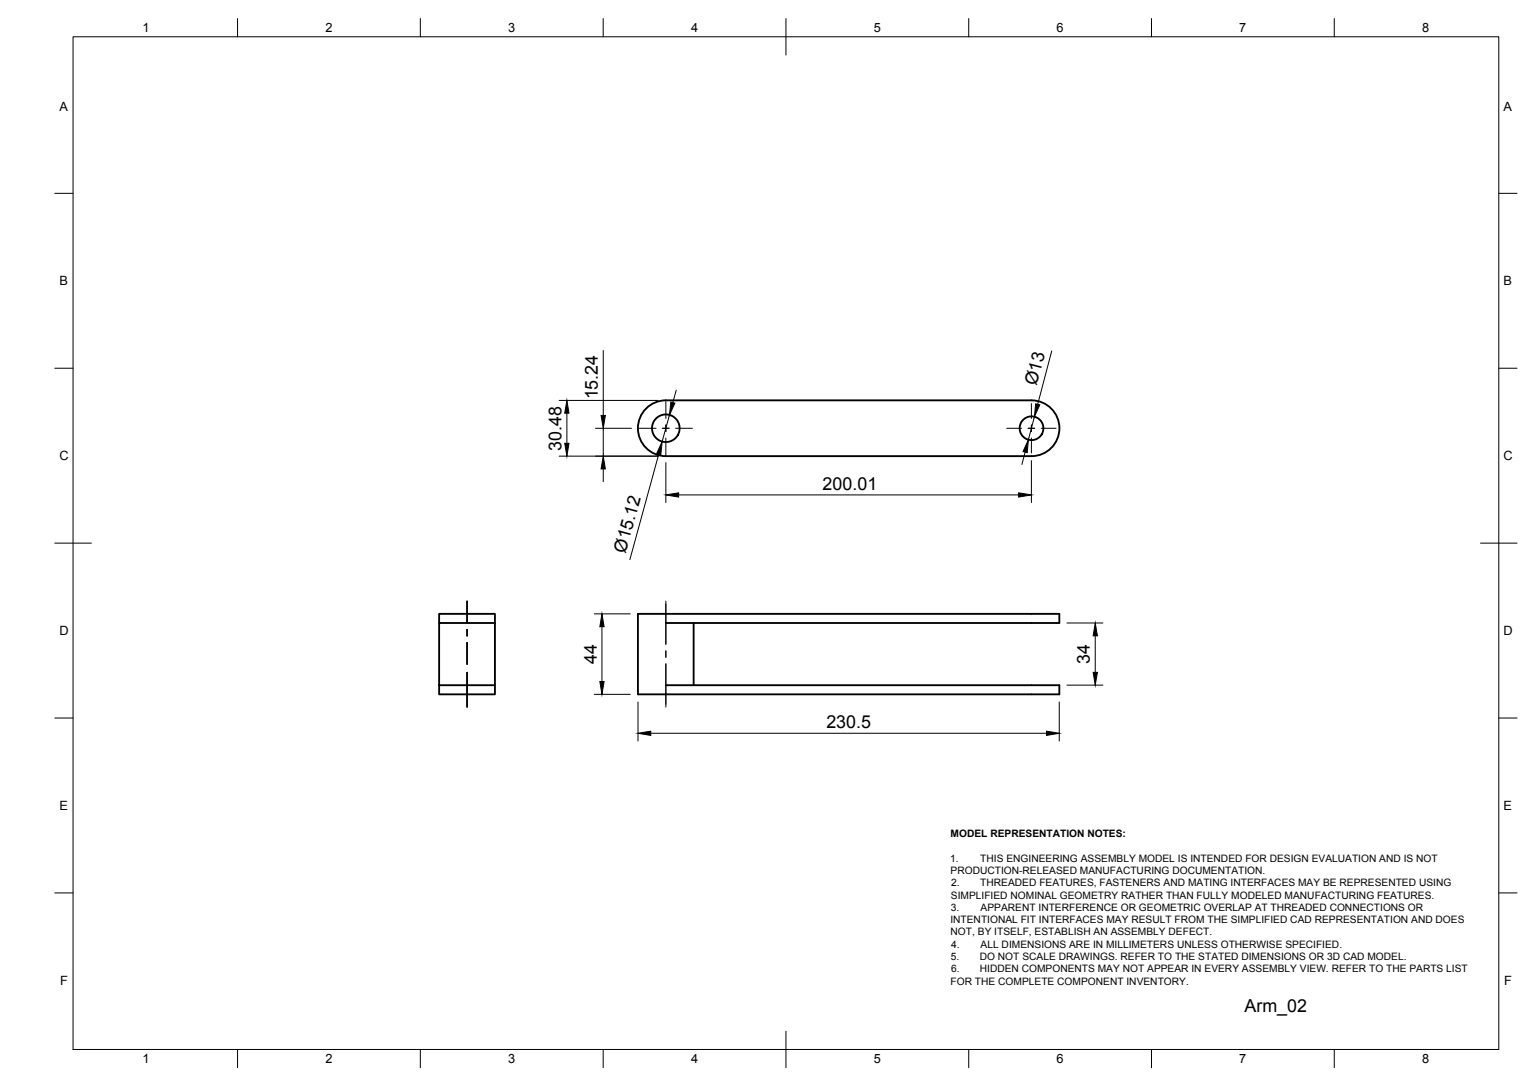
ISO-10303-21;
HEADER;
/* Generated by software containing ST-Developer
 * from STEP Tools, Inc. (www.steptools.com) 
 */

FILE_DESCRIPTION(
/* description */ (''),
/* implementation_level */ '2;1');

FILE_NAME(
/* name */ 'Arm_02.step',
/* time_stamp */ '2026-10-06T13:41:14-07:00',
/* author */ (''),
/* organization */ (''),
/* preprocessor_version */ 'ST-DEVELOPER v20.2',
/* originating_system */ 'Autodesk Translation Framework v15.15.0.0',
/* authorisation */ '');

FILE_SCHEMA (('AUTOMOTIVE_DESIGN { 1 0 10303 214 3 1 1 }'));
ENDSEC;

DATA;
#10=MECHANICAL_DESIGN_GEOMETRIC_PRESENTATION_REPRESENTATION('',(#1968),#279266);
#1950=SHAPE_REPRESENTATION_RELATIONSHIP('SRR','None',#279309,#1959);
#1959=ADVANCED_BREP_SHAPE_REPRESENTATION('',(#1977),#279265);
#1968=STYLED_ITEM('',(#279355),#1977);
#1977=MANIFOLD_SOLID_BREP('Body1',#14946);
#2018=FACE_BOUND('',#3081,.T.);
#2019=FACE_BOUND('',#3083,.T.);
#2020=FACE_BOUND('',#3084,.T.);
#2021=FACE_BOUND('',#3092,.T.);
#2022=FACE_BOUND('',#3094,.T.);
#2023=FACE_BOUND('',#3095,.T.);
#2102=PLANE('',#15640);
#2103=PLANE('',#15644);
#2104=PLANE('',#15645);
#2105=PLANE('',#15647);
#2106=PLANE('',#15655);
#2107=PLANE('',#15659);
#2108=PLANE('',#15663);
#2109=PLANE('',#15664);
#2566=FACE_OUTER_BOUND('',#3076,.T.);
#2567=FACE_OUTER_BOUND('',#3077,.T.);
#2568=FACE_OUTER_BOUND('',#3078,.T.);
#2569=FACE_OUTER_BOUND('',#3079,.T.);
#2570=FACE_OUTER_BOUND('',#3080,.T.);
#2571=FACE_OUTER_BOUND('',#3082,.T.);
#2572=FACE_OUTER_BOUND('',#3085,.T.);
#2573=FACE_OUTER_BOUND('',#3086,.T.);
#2574=FACE_OUTER_BOUND('',#3087,.T.);
#2575=FACE_OUTER_BOUND('',#3088,.T.);
#2576=FACE_OUTER_BOUND('',#3089,.T.);
#2577=FACE_OUTER_BOUND('',#3090,.T.);
#2578=FACE_OUTER_BOUND('',#3091,.T.);
#2579=FACE_OUTER_BOUND('',#3093,.T.);
#3076=EDGE_LOOP('',(#14026,#14027,#14028,#14029));
#3077=EDGE_LOOP('',(#14030,#14031,#14032,#14033));
#3078=EDGE_LOOP('',(#14034,#14035,#14036,#14037));
#3079=EDGE_LOOP('',(#14038,#14039,#14040,#14041));
#3080=EDGE_LOOP('',(#14042,#14043,#14044,#14045));
#3081=EDGE_LOOP('',(#14046));
#3082=EDGE_LOOP('',(#14047,#14048,#14049,#14050));
#3083=EDGE_LOOP('',(#14051));
#3084=EDGE_LOOP('',(#14052));
#3085=EDGE_LOOP('',(#14053,#14054,#14055,#14056));
#3086=EDGE_LOOP('',(#14057,#14058,#14059,#14060));
#3087=EDGE_LOOP('',(#14061,#14062,#14063,#14064));
#3088=EDGE_LOOP('',(#14065,#14066,#14067,#14068));
#3089=EDGE_LOOP('',(#14069,#14070,#14071,#14072));
#3090=EDGE_LOOP('',(#14073,#14074,#14075,#14076,#14077,#14078,#14079,#14080,
#14081,#14082));
#3091=EDGE_LOOP('',(#14083,#14084,#14085,#14086));
#3092=EDGE_LOOP('',(#14087));
#3093=EDGE_LOOP('',(#14088,#14089,#14090,#14091));
#3094=EDGE_LOOP('',(#14092));
#3095=EDGE_LOOP('',(#14093));
#3604=LINE('',#279170,#4132);
#3605=LINE('',#279175,#4133);
#3606=LINE('',#279177,#4134);
#3607=LINE('',#279179,#4135);
#3608=LINE('',#279180,#4136);
#3609=LINE('',#279186,#4137);
#3610=LINE('',#279189,#4138);
#3611=LINE('',#279191,#4139);
#3612=LINE('',#279192,#4140);
#3613=LINE('',#279201,#4141);
#3614=LINE('',#279207,#4142);
#3615=LINE('',#279212,#4143);
#3616=LINE('',#279214,#4144);
#3617=LINE('',#279216,#4145);
#3618=LINE('',#279217,#4146);
#3619=LINE('',#279222,#4147);
#3620=LINE('',#279226,#4148);
#3621=LINE('',#279228,#4149);
#3622=LINE('',#279229,#4150);
#3623=LINE('',#279233,#4151);
#4132=VECTOR('',#17366,6.50110764916953);
#4133=VECTOR('',#17371,10.);
#4134=VECTOR('',#17372,10.);
#4135=VECTOR('',#17373,10.);
#4136=VECTOR('',#17374,10.);
#4137=VECTOR('',#17381,10.);
#4138=VECTOR('',#17384,10.);
#4139=VECTOR('',#17385,10.);
#4140=VECTOR('',#17386,10.);
#4141=VECTOR('',#17399,7.55784864301595);
#4142=VECTOR('',#17406,6.50110764916953);
#4143=VECTOR('',#17411,10.);
#4144=VECTOR('',#17412,10.);
#4145=VECTOR('',#17413,10.);
#4146=VECTOR('',#17414,10.);
#4147=VECTOR('',#17419,10.);
#4148=VECTOR('',#17424,10.);
#4149=VECTOR('',#17425,10.);
#4150=VECTOR('',#17426,10.);
#4151=VECTOR('',#17433,15.2420394990918);
#4286=CIRCLE('',#15638,6.50110764916953);
#4287=CIRCLE('',#15639,6.50110764916953);
#4288=CIRCLE('',#15642,15.2420394990918);
#4289=CIRCLE('',#15643,15.2420394990918);
#4290=CIRCLE('',#15646,15.2420394990918);
#4291=CIRCLE('',#15648,15.2420394990918);
#4292=CIRCLE('',#15649,7.55784864301595);
#4293=CIRCLE('',#15651,7.55784864301595);
#4294=CIRCLE('',#15653,6.50110764916953);
#4295=CIRCLE('',#15654,6.50110764916953);
#4296=CIRCLE('',#15657,15.2420394990918);
#4297=CIRCLE('',#15658,15.2420394990918);
#4298=CIRCLE('',#15661,15.2420394990918);
#4299=CIRCLE('',#15662,15.2420394990918);
#6389=VERTEX_POINT('',#279167);
#6390=VERTEX_POINT('',#279169);
#6391=VERTEX_POINT('',#279173);
#6392=VERTEX_POINT('',#279174);
#6393=VERTEX_POINT('',#279176);
#6394=VERTEX_POINT('',#279178);
#6395=VERTEX_POINT('',#279182);
#6396=VERTEX_POINT('',#279184);
#6397=VERTEX_POINT('',#279188);
#6398=VERTEX_POINT('',#279190);
#6399=VERTEX_POINT('',#279197);
#6400=VERTEX_POINT('',#279200);
#6401=VERTEX_POINT('',#279204);
#6402=VERTEX_POINT('',#279206);
#6403=VERTEX_POINT('',#279210);
#6404=VERTEX_POINT('',#279211);
#6405=VERTEX_POINT('',#279213);
#6406=VERTEX_POINT('',#279215);
#6407=VERTEX_POINT('',#279219);
#6408=VERTEX_POINT('',#279221);
#6409=VERTEX_POINT('',#279225);
#6410=VERTEX_POINT('',#279227);
#8938=EDGE_CURVE('',#6389,#6389,#4286,.T.);
#8939=EDGE_CURVE('',#6389,#6390,#3604,.T.);
#8940=EDGE_CURVE('',#6390,#6390,#4287,.T.);
#8941=EDGE_CURVE('',#6391,#6392,#3605,.T.);
#8942=EDGE_CURVE('',#6392,#6393,#3606,.T.);
#8943=EDGE_CURVE('',#6394,#6393,#3607,.T.);
#8944=EDGE_CURVE('',#6391,#6394,#3608,.T.);
#8945=EDGE_CURVE('',#6395,#6391,#4288,.T.);
#8946=EDGE_CURVE('',#6396,#6394,#4289,.T.);
#8947=EDGE_CURVE('',#6395,#6396,#3609,.T.);
#8948=EDGE_CURVE('',#6397,#6395,#3610,.T.);
#8949=EDGE_CURVE('',#6398,#6396,#3611,.T.);
#8950=EDGE_CURVE('',#6397,#6398,#3612,.T.);
#8951=EDGE_CURVE('',#6393,#6398,#4290,.T.);
#8952=EDGE_CURVE('',#6392,#6397,#4291,.T.);
#8953=EDGE_CURVE('',#6399,#6399,#4292,.T.);
#8954=EDGE_CURVE('',#6399,#6400,#3613,.T.);
#8955=EDGE_CURVE('',#6400,#6400,#4293,.T.);
#8956=EDGE_CURVE('',#6401,#6401,#4294,.T.);
#8957=EDGE_CURVE('',#6401,#6402,#3614,.T.);
#8958=EDGE_CURVE('',#6402,#6402,#4295,.T.);
#8959=EDGE_CURVE('',#6403,#6404,#3615,.T.);
#8960=EDGE_CURVE('',#6403,#6405,#3616,.T.);
#8961=EDGE_CURVE('',#6405,#6406,#3617,.T.);
#8962=EDGE_CURVE('',#6404,#6406,#3618,.T.);
#8963=EDGE_CURVE('',#6407,#6403,#4296,.T.);
#8964=EDGE_CURVE('',#6407,#6408,#3619,.T.);
#8965=EDGE_CURVE('',#6408,#6405,#4297,.T.);
#8966=EDGE_CURVE('',#6409,#6407,#3620,.T.);
#8967=EDGE_CURVE('',#6409,#6410,#3621,.T.);
#8968=EDGE_CURVE('',#6410,#6408,#3622,.T.);
#8969=EDGE_CURVE('',#6404,#6409,#4298,.T.);
#8970=EDGE_CURVE('',#6410,#6406,#4299,.T.);
#8971=EDGE_CURVE('',#6410,#6398,#3623,.T.);
#14026=ORIENTED_EDGE('',*,*,#8938,.T.);
#14027=ORIENTED_EDGE('',*,*,#8939,.T.);
#14028=ORIENTED_EDGE('',*,*,#8940,.F.);
#14029=ORIENTED_EDGE('',*,*,#8939,.F.);
#14030=ORIENTED_EDGE('',*,*,#8941,.T.);
#14031=ORIENTED_EDGE('',*,*,#8942,.T.);
#14032=ORIENTED_EDGE('',*,*,#8943,.F.);
#14033=ORIENTED_EDGE('',*,*,#8944,.F.);
#14034=ORIENTED_EDGE('',*,*,#8945,.T.);
#14035=ORIENTED_EDGE('',*,*,#8944,.T.);
#14036=ORIENTED_EDGE('',*,*,#8946,.F.);
#14037=ORIENTED_EDGE('',*,*,#8947,.F.);
#14038=ORIENTED_EDGE('',*,*,#8948,.T.);
#14039=ORIENTED_EDGE('',*,*,#8947,.T.);
#14040=ORIENTED_EDGE('',*,*,#8949,.F.);
#14041=ORIENTED_EDGE('',*,*,#8950,.F.);
#14042=ORIENTED_EDGE('',*,*,#8951,.T.);
#14043=ORIENTED_EDGE('',*,*,#8949,.T.);
#14044=ORIENTED_EDGE('',*,*,#8946,.T.);
#14045=ORIENTED_EDGE('',*,*,#8943,.T.);
#14046=ORIENTED_EDGE('',*,*,#8940,.T.);
#14047=ORIENTED_EDGE('',*,*,#8952,.F.);
#14048=ORIENTED_EDGE('',*,*,#8941,.F.);
#14049=ORIENTED_EDGE('',*,*,#8945,.F.);
#14050=ORIENTED_EDGE('',*,*,#8948,.F.);
#14051=ORIENTED_EDGE('',*,*,#8938,.F.);
#14052=ORIENTED_EDGE('',*,*,#8953,.F.);
#14053=ORIENTED_EDGE('',*,*,#8953,.T.);
#14054=ORIENTED_EDGE('',*,*,#8954,.T.);
#14055=ORIENTED_EDGE('',*,*,#8955,.F.);
#14056=ORIENTED_EDGE('',*,*,#8954,.F.);
#14057=ORIENTED_EDGE('',*,*,#8956,.T.);
#14058=ORIENTED_EDGE('',*,*,#8957,.T.);
#14059=ORIENTED_EDGE('',*,*,#8958,.F.);
#14060=ORIENTED_EDGE('',*,*,#8957,.F.);
#14061=ORIENTED_EDGE('',*,*,#8959,.F.);
#14062=ORIENTED_EDGE('',*,*,#8960,.T.);
#14063=ORIENTED_EDGE('',*,*,#8961,.T.);
#14064=ORIENTED_EDGE('',*,*,#8962,.F.);
#14065=ORIENTED_EDGE('',*,*,#8963,.F.);
#14066=ORIENTED_EDGE('',*,*,#8964,.T.);
#14067=ORIENTED_EDGE('',*,*,#8965,.T.);
#14068=ORIENTED_EDGE('',*,*,#8960,.F.);
#14069=ORIENTED_EDGE('',*,*,#8966,.F.);
#14070=ORIENTED_EDGE('',*,*,#8967,.T.);
#14071=ORIENTED_EDGE('',*,*,#8968,.T.);
#14072=ORIENTED_EDGE('',*,*,#8964,.F.);
#14073=ORIENTED_EDGE('',*,*,#8967,.F.);
#14074=ORIENTED_EDGE('',*,*,#8969,.F.);
#14075=ORIENTED_EDGE('',*,*,#8962,.T.);
#14076=ORIENTED_EDGE('',*,*,#8970,.F.);
#14077=ORIENTED_EDGE('',*,*,#8971,.T.);
#14078=ORIENTED_EDGE('',*,*,#8951,.F.);
#14079=ORIENTED_EDGE('',*,*,#8942,.F.);
#14080=ORIENTED_EDGE('',*,*,#8952,.T.);
#14081=ORIENTED_EDGE('',*,*,#8950,.T.);
#14082=ORIENTED_EDGE('',*,*,#8971,.F.);
#14083=ORIENTED_EDGE('',*,*,#8970,.T.);
#14084=ORIENTED_EDGE('',*,*,#8961,.F.);
#14085=ORIENTED_EDGE('',*,*,#8965,.F.);
#14086=ORIENTED_EDGE('',*,*,#8968,.F.);
#14087=ORIENTED_EDGE('',*,*,#8956,.F.);
#14088=ORIENTED_EDGE('',*,*,#8969,.T.);
#14089=ORIENTED_EDGE('',*,*,#8966,.T.);
#14090=ORIENTED_EDGE('',*,*,#8963,.T.);
#14091=ORIENTED_EDGE('',*,*,#8959,.T.);
#14092=ORIENTED_EDGE('',*,*,#8958,.T.);
#14093=ORIENTED_EDGE('',*,*,#8955,.T.);
#14462=CYLINDRICAL_SURFACE('',#15637,6.50110764916953);
#14463=CYLINDRICAL_SURFACE('',#15641,15.2420394990918);
#14464=CYLINDRICAL_SURFACE('',#15650,7.55784864301595);
#14465=CYLINDRICAL_SURFACE('',#15652,6.50110764916953);
#14466=CYLINDRICAL_SURFACE('',#15656,15.2420394990918);
#14467=CYLINDRICAL_SURFACE('',#15660,15.2420394990918);
#14924=ADVANCED_FACE('',(#2566),#14462,.F.);
#14925=ADVANCED_FACE('',(#2567),#2102,.T.);
#14926=ADVANCED_FACE('',(#2568),#14463,.T.);
#14927=ADVANCED_FACE('',(#2569),#2103,.T.);
#14928=ADVANCED_FACE('',(#2570,#2018),#2104,.T.);
#14929=ADVANCED_FACE('',(#2571,#2019,#2020),#2105,.F.);
#14930=ADVANCED_FACE('',(#2572),#14464,.F.);
#14931=ADVANCED_FACE('',(#2573),#14465,.F.);
#14932=ADVANCED_FACE('',(#2574),#2106,.F.);
#14933=ADVANCED_FACE('',(#2575),#14466,.T.);
#14934=ADVANCED_FACE('',(#2576),#2107,.F.);
#14935=ADVANCED_FACE('',(#2577),#14467,.T.);
#14936=ADVANCED_FACE('',(#2578,#2021),#2108,.F.);
#14937=ADVANCED_FACE('',(#2579,#2022,#2023),#2109,.T.);
#14946=CLOSED_SHELL('',(#14924,#14925,#14926,#14927,#14928,#14929,#14930,
#14931,#14932,#14933,#14934,#14935,#14936,#14937));
#15636=AXIS2_PLACEMENT_3D('',#279165,#17360,#17361);
#15637=AXIS2_PLACEMENT_3D('',#279166,#17362,#17363);
#15638=AXIS2_PLACEMENT_3D('',#279168,#17364,#17365);
#15639=AXIS2_PLACEMENT_3D('',#279171,#17367,#17368);
#15640=AXIS2_PLACEMENT_3D('',#279172,#17369,#17370);
#15641=AXIS2_PLACEMENT_3D('',#279181,#17375,#17376);
#15642=AXIS2_PLACEMENT_3D('',#279183,#17377,#17378);
#15643=AXIS2_PLACEMENT_3D('',#279185,#17379,#17380);
#15644=AXIS2_PLACEMENT_3D('',#279187,#17382,#17383);
#15645=AXIS2_PLACEMENT_3D('',#279193,#17387,#17388);
#15646=AXIS2_PLACEMENT_3D('',#279194,#17389,#17390);
#15647=AXIS2_PLACEMENT_3D('',#279195,#17391,#17392);
#15648=AXIS2_PLACEMENT_3D('',#279196,#17393,#17394);
#15649=AXIS2_PLACEMENT_3D('',#279198,#17395,#17396);
#15650=AXIS2_PLACEMENT_3D('',#279199,#17397,#17398);
#15651=AXIS2_PLACEMENT_3D('',#279202,#17400,#17401);
#15652=AXIS2_PLACEMENT_3D('',#279203,#17402,#17403);
#15653=AXIS2_PLACEMENT_3D('',#279205,#17404,#17405);
#15654=AXIS2_PLACEMENT_3D('',#279208,#17407,#17408);
#15655=AXIS2_PLACEMENT_3D('',#279209,#17409,#17410);
#15656=AXIS2_PLACEMENT_3D('',#279218,#17415,#17416);
#15657=AXIS2_PLACEMENT_3D('',#279220,#17417,#17418);
#15658=AXIS2_PLACEMENT_3D('',#279223,#17420,#17421);
#15659=AXIS2_PLACEMENT_3D('',#279224,#17422,#17423);
#15660=AXIS2_PLACEMENT_3D('',#279230,#17427,#17428);
#15661=AXIS2_PLACEMENT_3D('',#279231,#17429,#17430);
#15662=AXIS2_PLACEMENT_3D('',#279232,#17431,#17432);
#15663=AXIS2_PLACEMENT_3D('',#279234,#17434,#17435);
#15664=AXIS2_PLACEMENT_3D('',#279235,#17436,#17437);
#17360=DIRECTION('axis',(0.,0.,1.));
#17361=DIRECTION('refdir',(1.,0.,0.));
#17362=DIRECTION('center_axis',(0.,-1.,0.));
#17363=DIRECTION('ref_axis',(-1.,0.,0.));
#17364=DIRECTION('center_axis',(0.,1.,0.));
#17365=DIRECTION('ref_axis',(-1.,0.,0.));
#17366=DIRECTION('',(0.,-1.,0.));
#17367=DIRECTION('center_axis',(0.,1.,0.));
#17368=DIRECTION('ref_axis',(-1.,0.,0.));
#17369=DIRECTION('center_axis',(-0.504104280893361,0.,-0.863642793048716));
#17370=DIRECTION('ref_axis',(0.863642793048716,0.,-0.504104280893361));
#17371=DIRECTION('',(0.863642793048716,0.,-0.504104280893361));
#17372=DIRECTION('',(0.,-1.,0.));
#17373=DIRECTION('',(0.863642793048716,0.,-0.504104280893361));
#17374=DIRECTION('',(0.,-1.,0.));
#17375=DIRECTION('center_axis',(0.,-1.,0.));
#17376=DIRECTION('ref_axis',(0.504104280893359,0.,0.863642793048717));
#17377=DIRECTION('center_axis',(0.,-1.,0.));
#17378=DIRECTION('ref_axis',(0.504104280893359,0.,0.863642793048717));
#17379=DIRECTION('center_axis',(0.,-1.,0.));
#17380=DIRECTION('ref_axis',(0.504104280893359,0.,0.863642793048717));
#17381=DIRECTION('',(0.,-1.,0.));
#17382=DIRECTION('center_axis',(0.504104280893361,0.,0.863642793048716));
#17383=DIRECTION('ref_axis',(-0.863642793048716,0.,0.504104280893361));
#17384=DIRECTION('',(-0.863642793048716,0.,0.504104280893361));
#17385=DIRECTION('',(-0.863642793048716,0.,0.504104280893361));
#17386=DIRECTION('',(0.,-1.,0.));
#17387=DIRECTION('center_axis',(0.,-1.,0.));
#17388=DIRECTION('ref_axis',(-1.,0.,0.));
#17389=DIRECTION('center_axis',(0.,1.,0.));
#17390=DIRECTION('ref_axis',(-1.,0.,0.));
#17391=DIRECTION('center_axis',(0.,-1.,0.));
#17392=DIRECTION('ref_axis',(-1.,0.,0.));
#17393=DIRECTION('center_axis',(0.,-1.,0.));
#17394=DIRECTION('ref_axis',(-0.50410428089336,0.,-0.863642793048716));
#17395=DIRECTION('center_axis',(-2.43566064310008E-53,1.,-1.62748695315959E-104));
#17396=DIRECTION('ref_axis',(-1.,-2.43566064310008E-53,0.));
#17397=DIRECTION('center_axis',(0.,-1.,0.));
#17398=DIRECTION('ref_axis',(-1.,0.,0.));
#17399=DIRECTION('',(0.,-1.,0.));
#17400=DIRECTION('center_axis',(2.43566064310008E-53,1.,1.62748695315959E-104));
#17401=DIRECTION('ref_axis',(-1.,2.43566064310008E-53,0.));
#17402=DIRECTION('center_axis',(0.,-1.,0.));
#17403=DIRECTION('ref_axis',(-1.,0.,0.));
#17404=DIRECTION('center_axis',(0.,1.,0.));
#17405=DIRECTION('ref_axis',(-1.,0.,0.));
#17406=DIRECTION('',(0.,-1.,0.));
#17407=DIRECTION('center_axis',(0.,1.,0.));
#17408=DIRECTION('ref_axis',(-1.,0.,0.));
#17409=DIRECTION('center_axis',(0.504104280893361,0.,0.863642793048716));
#17410=DIRECTION('ref_axis',(0.863642793048716,0.,-0.504104280893361));
#17411=DIRECTION('',(0.863642793048716,0.,-0.504104280893361));
#17412=DIRECTION('',(0.,1.,0.));
#17413=DIRECTION('',(0.863642793048716,0.,-0.504104280893361));
#17414=DIRECTION('',(0.,1.,0.));
#17415=DIRECTION('center_axis',(0.,-1.,0.));
#17416=DIRECTION('ref_axis',(0.504104280893359,0.,0.863642793048717));
#17417=DIRECTION('center_axis',(0.,-1.,0.));
#17418=DIRECTION('ref_axis',(0.504104280893359,0.,0.863642793048717));
#17419=DIRECTION('',(0.,1.,0.));
#17420=DIRECTION('center_axis',(0.,-1.,0.));
#17421=DIRECTION('ref_axis',(0.504104280893359,0.,0.863642793048717));
#17422=DIRECTION('center_axis',(-0.504104280893361,0.,-0.863642793048716));
#17423=DIRECTION('ref_axis',(-0.863642793048716,0.,0.504104280893361));
#17424=DIRECTION('',(-0.863642793048716,0.,0.504104280893361));
#17425=DIRECTION('',(0.,1.,0.));
#17426=DIRECTION('',(-0.863642793048716,0.,0.504104280893361));
#17427=DIRECTION('center_axis',(0.,-1.,0.));
#17428=DIRECTION('ref_axis',(-0.50410428089336,0.,-0.863642793048716));
#17429=DIRECTION('center_axis',(0.,-1.,0.));
#17430=DIRECTION('ref_axis',(-0.50410428089336,0.,-0.863642793048716));
#17431=DIRECTION('center_axis',(0.,-1.,0.));
#17432=DIRECTION('ref_axis',(-1.,0.,0.));
#17433=DIRECTION('',(0.,1.,0.));
#17434=DIRECTION('center_axis',(0.,-1.,0.));
#17435=DIRECTION('ref_axis',(-1.,0.,0.));
#17436=DIRECTION('center_axis',(0.,-1.,0.));
#17437=DIRECTION('ref_axis',(-1.,0.,0.));
#279165=CARTESIAN_POINT('',(0.,0.,0.));
#279166=CARTESIAN_POINT('Origin',(-192.718407221598,22.,130.804360617566));
#279167=CARTESIAN_POINT('',(-186.217299572429,22.,130.804360617566));
#279168=CARTESIAN_POINT('Origin',(-192.718407221598,22.,130.804360617566));
#279169=CARTESIAN_POINT('',(-186.217299572429,17.,130.804360617566));
#279170=CARTESIAN_POINT('',(-186.217299572428,22.,130.804360617566));
#279171=CARTESIAN_POINT('Origin',(-192.718407221598,17.,130.804360617566));
#279172=CARTESIAN_POINT('Origin',(-200.401984582636,22.,117.640683052811));
#279173=CARTESIAN_POINT('',(-200.401984582636,22.,117.640683052811));
#279174=CARTESIAN_POINT('',(-27.6628184943316,22.,16.8136353382454));
#279175=CARTESIAN_POINT('',(-200.401984582636,22.,117.640683052811));
#279176=CARTESIAN_POINT('',(-27.6628184943316,17.,16.8136353382454));
#279177=CARTESIAN_POINT('',(-27.6628184943316,22.,16.8136353382454));
#279178=CARTESIAN_POINT('',(-200.401984582636,17.,117.640683052811));
#279179=CARTESIAN_POINT('',(-200.401984582636,17.,117.640683052811));
#279180=CARTESIAN_POINT('',(-200.401984582636,22.,117.640683052811));
#279181=CARTESIAN_POINT('Origin',(-192.718407221598,22.,130.804360617566));
#279182=CARTESIAN_POINT('',(-185.034829860561,22.,143.96803818232));
#279183=CARTESIAN_POINT('Origin',(-192.718407221598,22.,130.804360617566));
#279184=CARTESIAN_POINT('',(-185.034829860561,17.,143.96803818232));
#279185=CARTESIAN_POINT('Origin',(-192.718407221598,17.,130.804360617566));
#279186=CARTESIAN_POINT('',(-185.034829860561,22.,143.96803818232));
#279187=CARTESIAN_POINT('Origin',(-12.2956637722558,22.,43.1409904677544));
#279188=CARTESIAN_POINT('',(-12.2956637722558,22.,43.1409904677544));
#279189=CARTESIAN_POINT('',(-12.2956637722558,22.,43.1409904677544));
#279190=CARTESIAN_POINT('',(-12.2956637722558,17.,43.1409904677544));
#279191=CARTESIAN_POINT('',(-12.2956637722558,17.,43.1409904677544));
#279192=CARTESIAN_POINT('',(-12.2956637722558,22.,43.1409904677544));
#279193=CARTESIAN_POINT('Origin',(-106.348824177446,17.,80.3908367602827));
#279194=CARTESIAN_POINT('Origin',(-19.9792411332937,17.,29.9773129029999));
#279195=CARTESIAN_POINT('Origin',(-106.348824177446,22.,80.3908367602827));
#279196=CARTESIAN_POINT('Origin',(-19.9792411332937,22.,29.9773129029999));
#279197=CARTESIAN_POINT('',(-12.4213924902778,22.,29.9773129029999));
#279198=CARTESIAN_POINT('Origin',(-19.9792411332937,22.,29.9773129029999));
#279199=CARTESIAN_POINT('Origin',(-19.9792411332937,-22.,29.9773129029999));
#279200=CARTESIAN_POINT('',(-12.4213924902778,-22.,29.9773129029999));
#279201=CARTESIAN_POINT('',(-12.4213924902778,-22.,29.9773129029999));
#279202=CARTESIAN_POINT('Origin',(-19.9792411332937,-22.,29.9773129029999));
#279203=CARTESIAN_POINT('Origin',(-192.718407221598,-22.,130.804360617566));
#279204=CARTESIAN_POINT('',(-186.217299572429,-17.,130.804360617566));
#279205=CARTESIAN_POINT('Origin',(-192.718407221598,-17.,130.804360617566));
#279206=CARTESIAN_POINT('',(-186.217299572429,-22.,130.804360617566));
#279207=CARTESIAN_POINT('',(-186.217299572428,-22.,130.804360617566));
#279208=CARTESIAN_POINT('Origin',(-192.718407221598,-22.,130.804360617566));
#279209=CARTESIAN_POINT('Origin',(-200.401984582636,-22.,117.640683052811));
#279210=CARTESIAN_POINT('',(-200.401984582636,-22.,117.640683052811));
#279211=CARTESIAN_POINT('',(-27.6628184943316,-22.,16.8136353382454));
#279212=CARTESIAN_POINT('',(-200.401984582636,-22.,117.640683052811));
#279213=CARTESIAN_POINT('',(-200.401984582636,-17.,117.640683052811));
#279214=CARTESIAN_POINT('',(-200.401984582636,-22.,117.640683052811));
#279215=CARTESIAN_POINT('',(-27.6628184943316,-17.,16.8136353382454));
#279216=CARTESIAN_POINT('',(-200.401984582636,-17.,117.640683052811));
#279217=CARTESIAN_POINT('',(-27.6628184943316,-22.,16.8136353382454));
#279218=CARTESIAN_POINT('Origin',(-192.718407221598,-22.,130.804360617566));
#279219=CARTESIAN_POINT('',(-185.034829860561,-22.,143.96803818232));
#279220=CARTESIAN_POINT('Origin',(-192.718407221598,-22.,130.804360617566));
#279221=CARTESIAN_POINT('',(-185.034829860561,-17.,143.96803818232));
#279222=CARTESIAN_POINT('',(-185.034829860561,-22.,143.96803818232));
#279223=CARTESIAN_POINT('Origin',(-192.718407221598,-17.,130.804360617566));
#279224=CARTESIAN_POINT('Origin',(-12.2956637722558,-22.,43.1409904677544));
#279225=CARTESIAN_POINT('',(-12.2956637722558,-22.,43.1409904677544));
#279226=CARTESIAN_POINT('',(-12.2956637722558,-22.,43.1409904677544));
#279227=CARTESIAN_POINT('',(-12.2956637722558,-17.,43.1409904677544));
#279228=CARTESIAN_POINT('',(-12.2956637722558,-22.,43.1409904677544));
#279229=CARTESIAN_POINT('',(-12.2956637722558,-17.,43.1409904677544));
#279230=CARTESIAN_POINT('Origin',(-19.9792411332937,-22.,29.9773129029999));
#279231=CARTESIAN_POINT('Origin',(-19.9792411332937,-22.,29.9773129029999));
#279232=CARTESIAN_POINT('Origin',(-19.9792411332937,-17.,29.9773129029999));
#279233=CARTESIAN_POINT('',(-12.2956637722558,-22.,43.1409904677544));
#279234=CARTESIAN_POINT('Origin',(-106.348824177446,-17.,80.3908367602827));
#279235=CARTESIAN_POINT('Origin',(-106.348824177446,-22.,80.3908367602827));
#279254=UNCERTAINTY_MEASURE_WITH_UNIT(LENGTH_MEASURE(0.01),#279267,
'DISTANCE_ACCURACY_VALUE',
'Maximum model space distance between geometric entities at asserted c
onnectivities');
#279255=UNCERTAINTY_MEASURE_WITH_UNIT(LENGTH_MEASURE(0.01),#279267,
'DISTANCE_ACCURACY_VALUE',
'Maximum model space distance between geometric entities at asserted c
onnectivities');
#279265=(
GEOMETRIC_REPRESENTATION_CONTEXT(3)
GLOBAL_UNCERTAINTY_ASSIGNED_CONTEXT((#279254))
GLOBAL_UNIT_ASSIGNED_CONTEXT((#279267,#279269,#279270))
REPRESENTATION_CONTEXT('','3D')
);
#279266=(
GEOMETRIC_REPRESENTATION_CONTEXT(3)
GLOBAL_UNCERTAINTY_ASSIGNED_CONTEXT((#279255))
GLOBAL_UNIT_ASSIGNED_CONTEXT((#279267,#279269,#279270))
REPRESENTATION_CONTEXT('','3D')
);
#279267=(
LENGTH_UNIT()
NAMED_UNIT(*)
SI_UNIT(.MILLI.,.METRE.)
);
#279269=(
NAMED_UNIT(*)
PLANE_ANGLE_UNIT()
SI_UNIT($,.RADIAN.)
);
#279270=(
NAMED_UNIT(*)
SI_UNIT($,.STERADIAN.)
SOLID_ANGLE_UNIT()
);
#279280=SHAPE_DEFINITION_REPRESENTATION(#279290,#279309);
#279290=PRODUCT_DEFINITION_SHAPE('',$,#279320);
#279309=SHAPE_REPRESENTATION('',(#15636),#279265);
#279310=PRODUCT_DEFINITION_CONTEXT('part definition',#279342,'design');
#279320=PRODUCT_DEFINITION('Arm_02','Arm_02',#279330,#279310);
#279330=PRODUCT_DEFINITION_FORMATION('',$,#279353);
#279342=APPLICATION_CONTEXT(
'Core Data for Automotive Mechanical Design Process');
#279343=PRODUCT_CONTEXT('part definition',#279342,'mechanical');
#279353=PRODUCT('Arm_02','Arm_02',$,(#279343));
#279355=PRESENTATION_STYLE_ASSIGNMENT((#279357));
#279357=SURFACE_STYLE_USAGE(.BOTH.,#279359);
#279359=SURFACE_SIDE_STYLE('',(#279361));
#279361=SURFACE_STYLE_FILL_AREA(#279363);
#279363=FILL_AREA_STYLE('Opaque(160,160,160)',(#279365));
#279365=FILL_AREA_STYLE_COLOUR('Opaque(160,160,160)',#279367);
#279367=COLOUR_RGB('Opaque(160,160,160)', 0.66274510, 0.83137255, 0.94901961);
ENDSEC;
END-ISO-10303-21;
